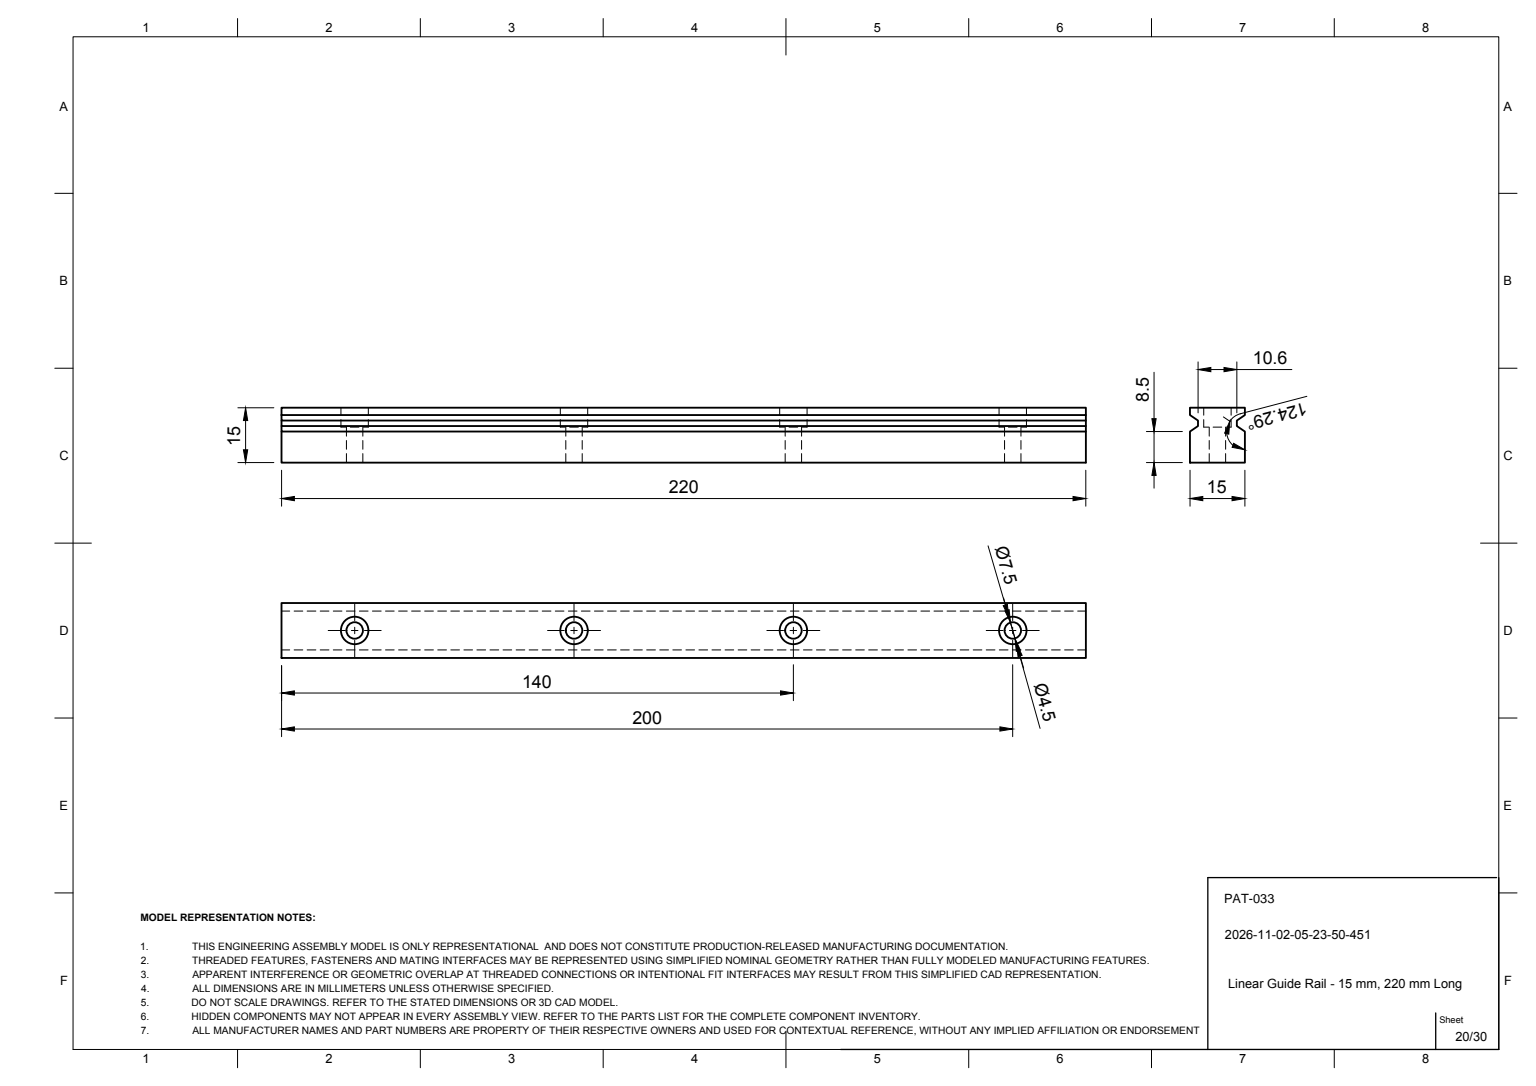
ISO-10303-21;
HEADER;
/* Generated by software containing ST-Developer
 * from STEP Tools, Inc. (www.steptools.com) 
 */

FILE_DESCRIPTION(
/* description */ ('Dual-rail gantry carriage'),
/* implementation_level */ '2;1');

FILE_NAME(
/* name */ 'Linear Guide Rail - 15 mm, 220 mm Long.step',
/* time_stamp */ '2026-10-27T10:49:15-07:00',
/* author */ (''),
/* organization */ (''),
/* preprocessor_version */ 'ST-DEVELOPER v20.2',
/* originating_system */ 'Autodesk Translation Framework v15.17.0.0',
/* authorisation */ '');

FILE_SCHEMA (('AUTOMOTIVE_DESIGN { 1 0 10303 214 3 1 1 }'));
ENDSEC;

DATA;
#10=MECHANICAL_DESIGN_GEOMETRIC_PRESENTATION_REPRESENTATION('',(#600),#12804);
#538=SHAPE_REPRESENTATION_RELATIONSHIP('SRR','None',#13016,#569);
#569=ADVANCED_BREP_SHAPE_REPRESENTATION('',(#631),#12786);
#600=STYLED_ITEM('',(#13240),#631);
#631=MANIFOLD_SOLID_BREP('Body1',#7378);
#692=FACE_BOUND('',#1660,.T.);
#693=FACE_BOUND('',#1663,.T.);
#694=FACE_BOUND('',#1666,.T.);
#695=FACE_BOUND('',#1669,.T.);
#696=FACE_BOUND('',#1679,.T.);
#697=FACE_BOUND('',#1680,.T.);
#698=FACE_BOUND('',#1681,.T.);
#699=FACE_BOUND('',#1682,.T.);
#700=FACE_BOUND('',#1689,.T.);
#701=FACE_BOUND('',#1690,.T.);
#702=FACE_BOUND('',#1691,.T.);
#703=FACE_BOUND('',#1692,.T.);
#902=PLANE('',#7999);
#903=PLANE('',#8004);
#904=PLANE('',#8009);
#905=PLANE('',#8014);
#906=PLANE('',#8024);
#907=PLANE('',#8025);
#908=PLANE('',#8026);
#909=PLANE('',#8027);
#910=PLANE('',#8028);
#911=PLANE('',#8029);
#912=PLANE('',#8030);
#913=PLANE('',#8031);
#914=PLANE('',#8032);
#915=PLANE('',#8033);
#916=PLANE('',#8034);
#917=PLANE('',#8035);
#918=PLANE('',#8036);
#919=PLANE('',#8037);
#1219=FACE_OUTER_BOUND('',#1658,.T.);
#1220=FACE_OUTER_BOUND('',#1659,.T.);
#1221=FACE_OUTER_BOUND('',#1661,.T.);
#1222=FACE_OUTER_BOUND('',#1662,.T.);
#1223=FACE_OUTER_BOUND('',#1664,.T.);
#1224=FACE_OUTER_BOUND('',#1665,.T.);
#1225=FACE_OUTER_BOUND('',#1667,.T.);
#1226=FACE_OUTER_BOUND('',#1668,.T.);
#1227=FACE_OUTER_BOUND('',#1670,.T.);
#1228=FACE_OUTER_BOUND('',#1671,.T.);
#1229=FACE_OUTER_BOUND('',#1672,.T.);
#1230=FACE_OUTER_BOUND('',#1673,.T.);
#1231=FACE_OUTER_BOUND('',#1674,.T.);
#1232=FACE_OUTER_BOUND('',#1675,.T.);
#1233=FACE_OUTER_BOUND('',#1676,.T.);
#1234=FACE_OUTER_BOUND('',#1677,.T.);
#1235=FACE_OUTER_BOUND('',#1678,.T.);
#1236=FACE_OUTER_BOUND('',#1683,.T.);
#1237=FACE_OUTER_BOUND('',#1684,.T.);
#1238=FACE_OUTER_BOUND('',#1685,.T.);
#1239=FACE_OUTER_BOUND('',#1686,.T.);
#1240=FACE_OUTER_BOUND('',#1687,.T.);
#1241=FACE_OUTER_BOUND('',#1688,.T.);
#1242=FACE_OUTER_BOUND('',#1693,.T.);
#1243=FACE_OUTER_BOUND('',#1694,.T.);
#1244=FACE_OUTER_BOUND('',#1695,.T.);
#1658=EDGE_LOOP('',(#5897,#5898,#5899,#5900));
#1659=EDGE_LOOP('',(#5901));
#1660=EDGE_LOOP('',(#5902));
#1661=EDGE_LOOP('',(#5903,#5904,#5905,#5906));
#1662=EDGE_LOOP('',(#5907));
#1663=EDGE_LOOP('',(#5908));
#1664=EDGE_LOOP('',(#5909,#5910,#5911,#5912));
#1665=EDGE_LOOP('',(#5913));
#1666=EDGE_LOOP('',(#5914));
#1667=EDGE_LOOP('',(#5915,#5916,#5917,#5918));
#1668=EDGE_LOOP('',(#5919));
#1669=EDGE_LOOP('',(#5920));
#1670=EDGE_LOOP('',(#5921,#5922,#5923,#5924));
#1671=EDGE_LOOP('',(#5925,#5926,#5927,#5928));
#1672=EDGE_LOOP('',(#5929,#5930,#5931,#5932));
#1673=EDGE_LOOP('',(#5933,#5934,#5935,#5936));
#1674=EDGE_LOOP('',(#5937,#5938,#5939,#5940));
#1675=EDGE_LOOP('',(#5941,#5942,#5943,#5944));
#1676=EDGE_LOOP('',(#5945,#5946,#5947,#5948));
#1677=EDGE_LOOP('',(#5949,#5950,#5951,#5952));
#1678=EDGE_LOOP('',(#5953,#5954,#5955,#5956));
#1679=EDGE_LOOP('',(#5957));
#1680=EDGE_LOOP('',(#5958));
#1681=EDGE_LOOP('',(#5959));
#1682=EDGE_LOOP('',(#5960));
#1683=EDGE_LOOP('',(#5961,#5962,#5963,#5964));
#1684=EDGE_LOOP('',(#5965,#5966,#5967,#5968));
#1685=EDGE_LOOP('',(#5969,#5970,#5971,#5972));
#1686=EDGE_LOOP('',(#5973,#5974,#5975,#5976));
#1687=EDGE_LOOP('',(#5977,#5978,#5979,#5980));
#1688=EDGE_LOOP('',(#5981,#5982,#5983,#5984));
#1689=EDGE_LOOP('',(#5985));
#1690=EDGE_LOOP('',(#5986));
#1691=EDGE_LOOP('',(#5987));
#1692=EDGE_LOOP('',(#5988));
#1693=EDGE_LOOP('',(#5989,#5990,#5991,#5992));
#1694=EDGE_LOOP('',(#5993,#5994,#5995,#5996,#5997,#5998,#5999,#6000,#6001,
#6002,#6003,#6004));
#1695=EDGE_LOOP('',(#6005,#6006,#6007,#6008,#6009,#6010,#6011,#6012,#6013,
#6014,#6015,#6016));
#2297=LINE('',#11562,#3006);
#2298=LINE('',#11571,#3007);
#2299=LINE('',#11580,#3008);
#2300=LINE('',#11589,#3009);
#2301=LINE('',#11597,#3010);
#2302=LINE('',#11601,#3011);
#2303=LINE('',#11605,#3012);
#2304=LINE('',#11609,#3013);
#2305=LINE('',#11613,#3014);
#2306=LINE('',#11615,#3015);
#2307=LINE('',#11617,#3016);
#2308=LINE('',#11618,#3017);
#2309=LINE('',#11621,#3018);
#2310=LINE('',#11623,#3019);
#2311=LINE('',#11624,#3020);
#2312=LINE('',#11627,#3021);
#2313=LINE('',#11629,#3022);
#2314=LINE('',#11630,#3023);
#2315=LINE('',#11633,#3024);
#2316=LINE('',#11635,#3025);
#2317=LINE('',#11636,#3026);
#2318=LINE('',#11639,#3027);
#2319=LINE('',#11641,#3028);
#2320=LINE('',#11642,#3029);
#2321=LINE('',#11645,#3030);
#2322=LINE('',#11647,#3031);
#2323=LINE('',#11648,#3032);
#2324=LINE('',#11651,#3033);
#2325=LINE('',#11653,#3034);
#2326=LINE('',#11654,#3035);
#2327=LINE('',#11657,#3036);
#2328=LINE('',#11659,#3037);
#2329=LINE('',#11660,#3038);
#2330=LINE('',#11663,#3039);
#2331=LINE('',#11665,#3040);
#2332=LINE('',#11666,#3041);
#2333=LINE('',#11669,#3042);
#2334=LINE('',#11671,#3043);
#2335=LINE('',#11672,#3044);
#2336=LINE('',#11675,#3045);
#2337=LINE('',#11677,#3046);
#2338=LINE('',#11678,#3047);
#2339=LINE('',#11680,#3048);
#2340=LINE('',#11681,#3049);
#3006=VECTOR('',#9350,0.375);
#3007=VECTOR('',#9361,0.375);
#3008=VECTOR('',#9372,0.375);
#3009=VECTOR('',#9383,0.375);
#3010=VECTOR('',#9394,0.225);
#3011=VECTOR('',#9399,0.225);
#3012=VECTOR('',#9404,0.225);
#3013=VECTOR('',#9409,0.225000000000001);
#3014=VECTOR('',#9412,1.);
#3015=VECTOR('',#9413,1.);
#3016=VECTOR('',#9414,1.);
#3017=VECTOR('',#9415,1.);
#3018=VECTOR('',#9418,1.);
#3019=VECTOR('',#9419,1.);
#3020=VECTOR('',#9420,1.);
#3021=VECTOR('',#9423,1.);
#3022=VECTOR('',#9424,1.);
#3023=VECTOR('',#9425,1.);
#3024=VECTOR('',#9428,1.);
#3025=VECTOR('',#9429,1.);
#3026=VECTOR('',#9430,1.);
#3027=VECTOR('',#9433,1.);
#3028=VECTOR('',#9434,1.);
#3029=VECTOR('',#9435,1.);
#3030=VECTOR('',#9438,1.);
#3031=VECTOR('',#9439,1.);
#3032=VECTOR('',#9440,1.);
#3033=VECTOR('',#9443,1.);
#3034=VECTOR('',#9444,1.);
#3035=VECTOR('',#9445,1.);
#3036=VECTOR('',#9448,1.);
#3037=VECTOR('',#9449,1.);
#3038=VECTOR('',#9450,1.);
#3039=VECTOR('',#9453,1.);
#3040=VECTOR('',#9454,1.);
#3041=VECTOR('',#9455,1.);
#3042=VECTOR('',#9458,1.);
#3043=VECTOR('',#9459,1.);
#3044=VECTOR('',#9460,1.);
#3045=VECTOR('',#9463,1.);
#3046=VECTOR('',#9464,1.);
#3047=VECTOR('',#9465,1.);
#3048=VECTOR('',#9468,1.);
#3049=VECTOR('',#9469,1.);
#3432=CIRCLE('',#7997,0.375);
#3433=CIRCLE('',#7998,0.375);
#3434=CIRCLE('',#8000,0.225);
#3435=CIRCLE('',#8002,0.375);
#3436=CIRCLE('',#8003,0.375);
#3437=CIRCLE('',#8005,0.225);
#3438=CIRCLE('',#8007,0.375);
#3439=CIRCLE('',#8008,0.375);
#3440=CIRCLE('',#8010,0.225);
#3441=CIRCLE('',#8012,0.375);
#3442=CIRCLE('',#8013,0.375);
#3443=CIRCLE('',#8015,0.225000000000001);
#3444=CIRCLE('',#8017,0.225);
#3445=CIRCLE('',#8019,0.225);
#3446=CIRCLE('',#8021,0.225);
#3447=CIRCLE('',#8023,0.225000000000001);
#3832=VERTEX_POINT('',#11559);
#3833=VERTEX_POINT('',#11561);
#3834=VERTEX_POINT('',#11565);
#3835=VERTEX_POINT('',#11568);
#3836=VERTEX_POINT('',#11570);
#3837=VERTEX_POINT('',#11574);
#3838=VERTEX_POINT('',#11577);
#3839=VERTEX_POINT('',#11579);
#3840=VERTEX_POINT('',#11583);
#3841=VERTEX_POINT('',#11586);
#3842=VERTEX_POINT('',#11588);
#3843=VERTEX_POINT('',#11592);
#3844=VERTEX_POINT('',#11595);
#3845=VERTEX_POINT('',#11599);
#3846=VERTEX_POINT('',#11603);
#3847=VERTEX_POINT('',#11607);
#3848=VERTEX_POINT('',#11611);
#3849=VERTEX_POINT('',#11612);
#3850=VERTEX_POINT('',#11614);
#3851=VERTEX_POINT('',#11616);
#3852=VERTEX_POINT('',#11620);
#3853=VERTEX_POINT('',#11622);
#3854=VERTEX_POINT('',#11626);
#3855=VERTEX_POINT('',#11628);
#3856=VERTEX_POINT('',#11632);
#3857=VERTEX_POINT('',#11634);
#3858=VERTEX_POINT('',#11638);
#3859=VERTEX_POINT('',#11640);
#3860=VERTEX_POINT('',#11644);
#3861=VERTEX_POINT('',#11646);
#3862=VERTEX_POINT('',#11650);
#3863=VERTEX_POINT('',#11652);
#3864=VERTEX_POINT('',#11656);
#3865=VERTEX_POINT('',#11658);
#3866=VERTEX_POINT('',#11662);
#3867=VERTEX_POINT('',#11664);
#3868=VERTEX_POINT('',#11668);
#3869=VERTEX_POINT('',#11670);
#3870=VERTEX_POINT('',#11674);
#3871=VERTEX_POINT('',#11676);
#4571=EDGE_CURVE('',#3832,#3832,#3432,.T.);
#4572=EDGE_CURVE('',#3832,#3833,#2297,.T.);
#4573=EDGE_CURVE('',#3833,#3833,#3433,.T.);
#4574=EDGE_CURVE('',#3834,#3834,#3434,.T.);
#4575=EDGE_CURVE('',#3835,#3835,#3435,.T.);
#4576=EDGE_CURVE('',#3835,#3836,#2298,.T.);
#4577=EDGE_CURVE('',#3836,#3836,#3436,.T.);
#4578=EDGE_CURVE('',#3837,#3837,#3437,.T.);
#4579=EDGE_CURVE('',#3838,#3838,#3438,.T.);
#4580=EDGE_CURVE('',#3838,#3839,#2299,.T.);
#4581=EDGE_CURVE('',#3839,#3839,#3439,.T.);
#4582=EDGE_CURVE('',#3840,#3840,#3440,.T.);
#4583=EDGE_CURVE('',#3841,#3841,#3441,.T.);
#4584=EDGE_CURVE('',#3841,#3842,#2300,.T.);
#4585=EDGE_CURVE('',#3842,#3842,#3442,.T.);
#4586=EDGE_CURVE('',#3843,#3843,#3443,.T.);
#4587=EDGE_CURVE('',#3844,#3844,#3444,.T.);
#4588=EDGE_CURVE('',#3844,#3834,#2301,.T.);
#4589=EDGE_CURVE('',#3845,#3845,#3445,.T.);
#4590=EDGE_CURVE('',#3845,#3837,#2302,.T.);
#4591=EDGE_CURVE('',#3846,#3846,#3446,.T.);
#4592=EDGE_CURVE('',#3846,#3840,#2303,.T.);
#4593=EDGE_CURVE('',#3847,#3847,#3447,.T.);
#4594=EDGE_CURVE('',#3847,#3843,#2304,.T.);
#4595=EDGE_CURVE('',#3848,#3849,#2305,.T.);
#4596=EDGE_CURVE('',#3849,#3850,#2306,.T.);
#4597=EDGE_CURVE('',#3851,#3850,#2307,.T.);
#4598=EDGE_CURVE('',#3848,#3851,#2308,.T.);
#4599=EDGE_CURVE('',#3852,#3848,#2309,.T.);
#4600=EDGE_CURVE('',#3853,#3851,#2310,.T.);
#4601=EDGE_CURVE('',#3852,#3853,#2311,.T.);
#4602=EDGE_CURVE('',#3854,#3852,#2312,.T.);
#4603=EDGE_CURVE('',#3855,#3853,#2313,.T.);
#4604=EDGE_CURVE('',#3854,#3855,#2314,.T.);
#4605=EDGE_CURVE('',#3856,#3854,#2315,.T.);
#4606=EDGE_CURVE('',#3857,#3855,#2316,.T.);
#4607=EDGE_CURVE('',#3856,#3857,#2317,.T.);
#4608=EDGE_CURVE('',#3858,#3856,#2318,.T.);
#4609=EDGE_CURVE('',#3859,#3857,#2319,.T.);
#4610=EDGE_CURVE('',#3858,#3859,#2320,.T.);
#4611=EDGE_CURVE('',#3860,#3858,#2321,.T.);
#4612=EDGE_CURVE('',#3861,#3859,#2322,.T.);
#4613=EDGE_CURVE('',#3860,#3861,#2323,.T.);
#4614=EDGE_CURVE('',#3862,#3860,#2324,.T.);
#4615=EDGE_CURVE('',#3863,#3861,#2325,.T.);
#4616=EDGE_CURVE('',#3862,#3863,#2326,.T.);
#4617=EDGE_CURVE('',#3864,#3862,#2327,.T.);
#4618=EDGE_CURVE('',#3865,#3863,#2328,.T.);
#4619=EDGE_CURVE('',#3864,#3865,#2329,.T.);
#4620=EDGE_CURVE('',#3866,#3864,#2330,.T.);
#4621=EDGE_CURVE('',#3867,#3865,#2331,.T.);
#4622=EDGE_CURVE('',#3866,#3867,#2332,.T.);
#4623=EDGE_CURVE('',#3868,#3866,#2333,.T.);
#4624=EDGE_CURVE('',#3869,#3867,#2334,.T.);
#4625=EDGE_CURVE('',#3868,#3869,#2335,.T.);
#4626=EDGE_CURVE('',#3870,#3868,#2336,.T.);
#4627=EDGE_CURVE('',#3871,#3869,#2337,.T.);
#4628=EDGE_CURVE('',#3870,#3871,#2338,.T.);
#4629=EDGE_CURVE('',#3849,#3870,#2339,.T.);
#4630=EDGE_CURVE('',#3850,#3871,#2340,.T.);
#5897=ORIENTED_EDGE('',*,*,#4571,.F.);
#5898=ORIENTED_EDGE('',*,*,#4572,.T.);
#5899=ORIENTED_EDGE('',*,*,#4573,.F.);
#5900=ORIENTED_EDGE('',*,*,#4572,.F.);
#5901=ORIENTED_EDGE('',*,*,#4571,.T.);
#5902=ORIENTED_EDGE('',*,*,#4574,.F.);
#5903=ORIENTED_EDGE('',*,*,#4575,.F.);
#5904=ORIENTED_EDGE('',*,*,#4576,.T.);
#5905=ORIENTED_EDGE('',*,*,#4577,.F.);
#5906=ORIENTED_EDGE('',*,*,#4576,.F.);
#5907=ORIENTED_EDGE('',*,*,#4575,.T.);
#5908=ORIENTED_EDGE('',*,*,#4578,.F.);
#5909=ORIENTED_EDGE('',*,*,#4579,.F.);
#5910=ORIENTED_EDGE('',*,*,#4580,.T.);
#5911=ORIENTED_EDGE('',*,*,#4581,.F.);
#5912=ORIENTED_EDGE('',*,*,#4580,.F.);
#5913=ORIENTED_EDGE('',*,*,#4579,.T.);
#5914=ORIENTED_EDGE('',*,*,#4582,.F.);
#5915=ORIENTED_EDGE('',*,*,#4583,.F.);
#5916=ORIENTED_EDGE('',*,*,#4584,.T.);
#5917=ORIENTED_EDGE('',*,*,#4585,.F.);
#5918=ORIENTED_EDGE('',*,*,#4584,.F.);
#5919=ORIENTED_EDGE('',*,*,#4583,.T.);
#5920=ORIENTED_EDGE('',*,*,#4586,.F.);
#5921=ORIENTED_EDGE('',*,*,#4587,.F.);
#5922=ORIENTED_EDGE('',*,*,#4588,.T.);
#5923=ORIENTED_EDGE('',*,*,#4574,.T.);
#5924=ORIENTED_EDGE('',*,*,#4588,.F.);
#5925=ORIENTED_EDGE('',*,*,#4589,.F.);
#5926=ORIENTED_EDGE('',*,*,#4590,.T.);
#5927=ORIENTED_EDGE('',*,*,#4578,.T.);
#5928=ORIENTED_EDGE('',*,*,#4590,.F.);
#5929=ORIENTED_EDGE('',*,*,#4591,.F.);
#5930=ORIENTED_EDGE('',*,*,#4592,.T.);
#5931=ORIENTED_EDGE('',*,*,#4582,.T.);
#5932=ORIENTED_EDGE('',*,*,#4592,.F.);
#5933=ORIENTED_EDGE('',*,*,#4593,.F.);
#5934=ORIENTED_EDGE('',*,*,#4594,.T.);
#5935=ORIENTED_EDGE('',*,*,#4586,.T.);
#5936=ORIENTED_EDGE('',*,*,#4594,.F.);
#5937=ORIENTED_EDGE('',*,*,#4595,.T.);
#5938=ORIENTED_EDGE('',*,*,#4596,.T.);
#5939=ORIENTED_EDGE('',*,*,#4597,.F.);
#5940=ORIENTED_EDGE('',*,*,#4598,.F.);
#5941=ORIENTED_EDGE('',*,*,#4599,.T.);
#5942=ORIENTED_EDGE('',*,*,#4598,.T.);
#5943=ORIENTED_EDGE('',*,*,#4600,.F.);
#5944=ORIENTED_EDGE('',*,*,#4601,.F.);
#5945=ORIENTED_EDGE('',*,*,#4602,.T.);
#5946=ORIENTED_EDGE('',*,*,#4601,.T.);
#5947=ORIENTED_EDGE('',*,*,#4603,.F.);
#5948=ORIENTED_EDGE('',*,*,#4604,.F.);
#5949=ORIENTED_EDGE('',*,*,#4605,.T.);
#5950=ORIENTED_EDGE('',*,*,#4604,.T.);
#5951=ORIENTED_EDGE('',*,*,#4606,.F.);
#5952=ORIENTED_EDGE('',*,*,#4607,.F.);
#5953=ORIENTED_EDGE('',*,*,#4608,.T.);
#5954=ORIENTED_EDGE('',*,*,#4607,.T.);
#5955=ORIENTED_EDGE('',*,*,#4609,.F.);
#5956=ORIENTED_EDGE('',*,*,#4610,.F.);
#5957=ORIENTED_EDGE('',*,*,#4585,.T.);
#5958=ORIENTED_EDGE('',*,*,#4581,.T.);
#5959=ORIENTED_EDGE('',*,*,#4577,.T.);
#5960=ORIENTED_EDGE('',*,*,#4573,.T.);
#5961=ORIENTED_EDGE('',*,*,#4611,.T.);
#5962=ORIENTED_EDGE('',*,*,#4610,.T.);
#5963=ORIENTED_EDGE('',*,*,#4612,.F.);
#5964=ORIENTED_EDGE('',*,*,#4613,.F.);
#5965=ORIENTED_EDGE('',*,*,#4614,.T.);
#5966=ORIENTED_EDGE('',*,*,#4613,.T.);
#5967=ORIENTED_EDGE('',*,*,#4615,.F.);
#5968=ORIENTED_EDGE('',*,*,#4616,.F.);
#5969=ORIENTED_EDGE('',*,*,#4617,.T.);
#5970=ORIENTED_EDGE('',*,*,#4616,.T.);
#5971=ORIENTED_EDGE('',*,*,#4618,.F.);
#5972=ORIENTED_EDGE('',*,*,#4619,.F.);
#5973=ORIENTED_EDGE('',*,*,#4620,.T.);
#5974=ORIENTED_EDGE('',*,*,#4619,.T.);
#5975=ORIENTED_EDGE('',*,*,#4621,.F.);
#5976=ORIENTED_EDGE('',*,*,#4622,.F.);
#5977=ORIENTED_EDGE('',*,*,#4623,.T.);
#5978=ORIENTED_EDGE('',*,*,#4622,.T.);
#5979=ORIENTED_EDGE('',*,*,#4624,.F.);
#5980=ORIENTED_EDGE('',*,*,#4625,.F.);
#5981=ORIENTED_EDGE('',*,*,#4626,.T.);
#5982=ORIENTED_EDGE('',*,*,#4625,.T.);
#5983=ORIENTED_EDGE('',*,*,#4627,.F.);
#5984=ORIENTED_EDGE('',*,*,#4628,.F.);
#5985=ORIENTED_EDGE('',*,*,#4587,.T.);
#5986=ORIENTED_EDGE('',*,*,#4589,.T.);
#5987=ORIENTED_EDGE('',*,*,#4591,.T.);
#5988=ORIENTED_EDGE('',*,*,#4593,.T.);
#5989=ORIENTED_EDGE('',*,*,#4629,.T.);
#5990=ORIENTED_EDGE('',*,*,#4628,.T.);
#5991=ORIENTED_EDGE('',*,*,#4630,.F.);
#5992=ORIENTED_EDGE('',*,*,#4596,.F.);
#5993=ORIENTED_EDGE('',*,*,#4630,.T.);
#5994=ORIENTED_EDGE('',*,*,#4627,.T.);
#5995=ORIENTED_EDGE('',*,*,#4624,.T.);
#5996=ORIENTED_EDGE('',*,*,#4621,.T.);
#5997=ORIENTED_EDGE('',*,*,#4618,.T.);
#5998=ORIENTED_EDGE('',*,*,#4615,.T.);
#5999=ORIENTED_EDGE('',*,*,#4612,.T.);
#6000=ORIENTED_EDGE('',*,*,#4609,.T.);
#6001=ORIENTED_EDGE('',*,*,#4606,.T.);
#6002=ORIENTED_EDGE('',*,*,#4603,.T.);
#6003=ORIENTED_EDGE('',*,*,#4600,.T.);
#6004=ORIENTED_EDGE('',*,*,#4597,.T.);
#6005=ORIENTED_EDGE('',*,*,#4629,.F.);
#6006=ORIENTED_EDGE('',*,*,#4595,.F.);
#6007=ORIENTED_EDGE('',*,*,#4599,.F.);
#6008=ORIENTED_EDGE('',*,*,#4602,.F.);
#6009=ORIENTED_EDGE('',*,*,#4605,.F.);
#6010=ORIENTED_EDGE('',*,*,#4608,.F.);
#6011=ORIENTED_EDGE('',*,*,#4611,.F.);
#6012=ORIENTED_EDGE('',*,*,#4614,.F.);
#6013=ORIENTED_EDGE('',*,*,#4617,.F.);
#6014=ORIENTED_EDGE('',*,*,#4620,.F.);
#6015=ORIENTED_EDGE('',*,*,#4623,.F.);
#6016=ORIENTED_EDGE('',*,*,#4626,.F.);
#6922=CYLINDRICAL_SURFACE('',#7996,0.375);
#6923=CYLINDRICAL_SURFACE('',#8001,0.375);
#6924=CYLINDRICAL_SURFACE('',#8006,0.375);
#6925=CYLINDRICAL_SURFACE('',#8011,0.375);
#6926=CYLINDRICAL_SURFACE('',#8016,0.225);
#6927=CYLINDRICAL_SURFACE('',#8018,0.225);
#6928=CYLINDRICAL_SURFACE('',#8020,0.225);
#6929=CYLINDRICAL_SURFACE('',#8022,0.225000000000001);
#7145=ADVANCED_FACE('',(#1219),#6922,.F.);
#7146=ADVANCED_FACE('',(#1220,#692),#902,.T.);
#7147=ADVANCED_FACE('',(#1221),#6923,.F.);
#7148=ADVANCED_FACE('',(#1222,#693),#903,.T.);
#7149=ADVANCED_FACE('',(#1223),#6924,.F.);
#7150=ADVANCED_FACE('',(#1224,#694),#904,.T.);
#7151=ADVANCED_FACE('',(#1225),#6925,.F.);
#7152=ADVANCED_FACE('',(#1226,#695),#905,.T.);
#7153=ADVANCED_FACE('',(#1227),#6926,.F.);
#7154=ADVANCED_FACE('',(#1228),#6927,.F.);
#7155=ADVANCED_FACE('',(#1229),#6928,.F.);
#7156=ADVANCED_FACE('',(#1230),#6929,.F.);
#7157=ADVANCED_FACE('',(#1231),#906,.T.);
#7158=ADVANCED_FACE('',(#1232),#907,.T.);
#7159=ADVANCED_FACE('',(#1233),#908,.T.);
#7160=ADVANCED_FACE('',(#1234),#909,.T.);
#7161=ADVANCED_FACE('',(#1235,#696,#697,#698,#699),#910,.T.);
#7162=ADVANCED_FACE('',(#1236),#911,.T.);
#7163=ADVANCED_FACE('',(#1237),#912,.T.);
#7164=ADVANCED_FACE('',(#1238),#913,.T.);
#7165=ADVANCED_FACE('',(#1239),#914,.T.);
#7166=ADVANCED_FACE('',(#1240),#915,.T.);
#7167=ADVANCED_FACE('',(#1241,#700,#701,#702,#703),#916,.T.);
#7168=ADVANCED_FACE('',(#1242),#917,.T.);
#7169=ADVANCED_FACE('',(#1243),#918,.T.);
#7170=ADVANCED_FACE('',(#1244),#919,.F.);
#7378=CLOSED_SHELL('',(#7145,#7146,#7147,#7148,#7149,#7150,#7151,#7152,
#7153,#7154,#7155,#7156,#7157,#7158,#7159,#7160,#7161,#7162,#7163,#7164,
#7165,#7166,#7167,#7168,#7169,#7170));
#7995=AXIS2_PLACEMENT_3D('',#11557,#9344,#9345);
#7996=AXIS2_PLACEMENT_3D('',#11558,#9346,#9347);
#7997=AXIS2_PLACEMENT_3D('',#11560,#9348,#9349);
#7998=AXIS2_PLACEMENT_3D('',#11563,#9351,#9352);
#7999=AXIS2_PLACEMENT_3D('',#11564,#9353,#9354);
#8000=AXIS2_PLACEMENT_3D('',#11566,#9355,#9356);
#8001=AXIS2_PLACEMENT_3D('',#11567,#9357,#9358);
#8002=AXIS2_PLACEMENT_3D('',#11569,#9359,#9360);
#8003=AXIS2_PLACEMENT_3D('',#11572,#9362,#9363);
#8004=AXIS2_PLACEMENT_3D('',#11573,#9364,#9365);
#8005=AXIS2_PLACEMENT_3D('',#11575,#9366,#9367);
#8006=AXIS2_PLACEMENT_3D('',#11576,#9368,#9369);
#8007=AXIS2_PLACEMENT_3D('',#11578,#9370,#9371);
#8008=AXIS2_PLACEMENT_3D('',#11581,#9373,#9374);
#8009=AXIS2_PLACEMENT_3D('',#11582,#9375,#9376);
#8010=AXIS2_PLACEMENT_3D('',#11584,#9377,#9378);
#8011=AXIS2_PLACEMENT_3D('',#11585,#9379,#9380);
#8012=AXIS2_PLACEMENT_3D('',#11587,#9381,#9382);
#8013=AXIS2_PLACEMENT_3D('',#11590,#9384,#9385);
#8014=AXIS2_PLACEMENT_3D('',#11591,#9386,#9387);
#8015=AXIS2_PLACEMENT_3D('',#11593,#9388,#9389);
#8016=AXIS2_PLACEMENT_3D('',#11594,#9390,#9391);
#8017=AXIS2_PLACEMENT_3D('',#11596,#9392,#9393);
#8018=AXIS2_PLACEMENT_3D('',#11598,#9395,#9396);
#8019=AXIS2_PLACEMENT_3D('',#11600,#9397,#9398);
#8020=AXIS2_PLACEMENT_3D('',#11602,#9400,#9401);
#8021=AXIS2_PLACEMENT_3D('',#11604,#9402,#9403);
#8022=AXIS2_PLACEMENT_3D('',#11606,#9405,#9406);
#8023=AXIS2_PLACEMENT_3D('',#11608,#9407,#9408);
#8024=AXIS2_PLACEMENT_3D('',#11610,#9410,#9411);
#8025=AXIS2_PLACEMENT_3D('',#11619,#9416,#9417);
#8026=AXIS2_PLACEMENT_3D('',#11625,#9421,#9422);
#8027=AXIS2_PLACEMENT_3D('',#11631,#9426,#9427);
#8028=AXIS2_PLACEMENT_3D('',#11637,#9431,#9432);
#8029=AXIS2_PLACEMENT_3D('',#11643,#9436,#9437);
#8030=AXIS2_PLACEMENT_3D('',#11649,#9441,#9442);
#8031=AXIS2_PLACEMENT_3D('',#11655,#9446,#9447);
#8032=AXIS2_PLACEMENT_3D('',#11661,#9451,#9452);
#8033=AXIS2_PLACEMENT_3D('',#11667,#9456,#9457);
#8034=AXIS2_PLACEMENT_3D('',#11673,#9461,#9462);
#8035=AXIS2_PLACEMENT_3D('',#11679,#9466,#9467);
#8036=AXIS2_PLACEMENT_3D('',#11682,#9470,#9471);
#8037=AXIS2_PLACEMENT_3D('',#11683,#9472,#9473);
#9344=DIRECTION('axis',(0.,0.,1.));
#9345=DIRECTION('refdir',(1.,0.,0.));
#9346=DIRECTION('center_axis',(0.,0.,1.));
#9347=DIRECTION('ref_axis',(1.,0.,0.));
#9348=DIRECTION('center_axis',(0.,0.,1.));
#9349=DIRECTION('ref_axis',(1.,0.,0.));
#9350=DIRECTION('',(0.,0.,1.));
#9351=DIRECTION('center_axis',(0.,0.,-1.));
#9352=DIRECTION('ref_axis',(1.,0.,0.));
#9353=DIRECTION('center_axis',(0.,0.,1.));
#9354=DIRECTION('ref_axis',(1.,0.,0.));
#9355=DIRECTION('center_axis',(0.,0.,1.));
#9356=DIRECTION('ref_axis',(1.,0.,0.));
#9357=DIRECTION('center_axis',(0.,0.,1.));
#9358=DIRECTION('ref_axis',(1.,0.,0.));
#9359=DIRECTION('center_axis',(0.,0.,1.));
#9360=DIRECTION('ref_axis',(1.,0.,0.));
#9361=DIRECTION('',(0.,0.,1.));
#9362=DIRECTION('center_axis',(0.,0.,-1.));
#9363=DIRECTION('ref_axis',(1.,0.,0.));
#9364=DIRECTION('center_axis',(0.,0.,1.));
#9365=DIRECTION('ref_axis',(1.,0.,0.));
#9366=DIRECTION('center_axis',(0.,0.,1.));
#9367=DIRECTION('ref_axis',(1.,0.,0.));
#9368=DIRECTION('center_axis',(0.,0.,1.));
#9369=DIRECTION('ref_axis',(1.,0.,0.));
#9370=DIRECTION('center_axis',(0.,0.,1.));
#9371=DIRECTION('ref_axis',(1.,0.,0.));
#9372=DIRECTION('',(0.,0.,1.));
#9373=DIRECTION('center_axis',(0.,0.,-1.));
#9374=DIRECTION('ref_axis',(1.,0.,0.));
#9375=DIRECTION('center_axis',(0.,0.,1.));
#9376=DIRECTION('ref_axis',(1.,0.,0.));
#9377=DIRECTION('center_axis',(0.,0.,1.));
#9378=DIRECTION('ref_axis',(1.,0.,0.));
#9379=DIRECTION('center_axis',(0.,0.,1.));
#9380=DIRECTION('ref_axis',(1.,0.,0.));
#9381=DIRECTION('center_axis',(0.,0.,1.));
#9382=DIRECTION('ref_axis',(1.,0.,0.));
#9383=DIRECTION('',(0.,0.,1.));
#9384=DIRECTION('center_axis',(0.,0.,-1.));
#9385=DIRECTION('ref_axis',(1.,0.,0.));
#9386=DIRECTION('center_axis',(0.,0.,1.));
#9387=DIRECTION('ref_axis',(1.,0.,0.));
#9388=DIRECTION('center_axis',(0.,0.,1.));
#9389=DIRECTION('ref_axis',(1.,0.,0.));
#9390=DIRECTION('center_axis',(0.,0.,1.));
#9391=DIRECTION('ref_axis',(1.,0.,0.));
#9392=DIRECTION('center_axis',(0.,0.,1.));
#9393=DIRECTION('ref_axis',(1.,0.,0.));
#9394=DIRECTION('',(0.,0.,1.));
#9395=DIRECTION('center_axis',(0.,0.,1.));
#9396=DIRECTION('ref_axis',(1.,0.,0.));
#9397=DIRECTION('center_axis',(0.,0.,1.));
#9398=DIRECTION('ref_axis',(1.,0.,0.));
#9399=DIRECTION('',(0.,0.,1.));
#9400=DIRECTION('center_axis',(0.,0.,1.));
#9401=DIRECTION('ref_axis',(1.,0.,0.));
#9402=DIRECTION('center_axis',(0.,0.,1.));
#9403=DIRECTION('ref_axis',(1.,0.,0.));
#9404=DIRECTION('',(0.,0.,1.));
#9405=DIRECTION('center_axis',(0.,0.,1.));
#9406=DIRECTION('ref_axis',(1.,0.,0.));
#9407=DIRECTION('center_axis',(0.,0.,1.));
#9408=DIRECTION('ref_axis',(1.,0.,0.));
#9409=DIRECTION('',(0.,0.,1.));
#9410=DIRECTION('center_axis',(0.,-0.56333682464151,0.826227342807548));
#9411=DIRECTION('ref_axis',(0.,-0.826227342807548,-0.56333682464151));
#9412=DIRECTION('',(0.,-0.826227342807548,-0.56333682464151));
#9413=DIRECTION('',(1.,0.,0.));
#9414=DIRECTION('',(0.,-0.826227342807548,-0.56333682464151));
#9415=DIRECTION('',(1.,0.,0.));
#9416=DIRECTION('center_axis',(0.,-1.,0.));
#9417=DIRECTION('ref_axis',(0.,0.,-1.));
#9418=DIRECTION('',(0.,0.,-1.));
#9419=DIRECTION('',(0.,0.,-1.));
#9420=DIRECTION('',(1.,0.,0.));
#9421=DIRECTION('center_axis',(0.,-0.56333682464151,-0.826227342807548));
#9422=DIRECTION('ref_axis',(0.,0.826227342807548,-0.56333682464151));
#9423=DIRECTION('',(0.,0.826227342807548,-0.56333682464151));
#9424=DIRECTION('',(0.,0.826227342807548,-0.56333682464151));
#9425=DIRECTION('',(1.,0.,0.));
#9426=DIRECTION('center_axis',(0.,-1.,0.));
#9427=DIRECTION('ref_axis',(0.,0.,-1.));
#9428=DIRECTION('',(0.,0.,-1.));
#9429=DIRECTION('',(0.,0.,-1.));
#9430=DIRECTION('',(1.,0.,0.));
#9431=DIRECTION('center_axis',(0.,0.,1.));
#9432=DIRECTION('ref_axis',(0.,-1.,0.));
#9433=DIRECTION('',(0.,-1.,0.));
#9434=DIRECTION('',(0.,-1.,0.));
#9435=DIRECTION('',(1.,0.,0.));
#9436=DIRECTION('center_axis',(0.,1.,0.));
#9437=DIRECTION('ref_axis',(0.,0.,1.));
#9438=DIRECTION('',(0.,0.,1.));
#9439=DIRECTION('',(0.,0.,1.));
#9440=DIRECTION('',(1.,0.,0.));
#9441=DIRECTION('center_axis',(0.,0.56333682464151,-0.826227342807548));
#9442=DIRECTION('ref_axis',(0.,0.826227342807548,0.56333682464151));
#9443=DIRECTION('',(0.,0.826227342807548,0.56333682464151));
#9444=DIRECTION('',(0.,0.826227342807548,0.56333682464151));
#9445=DIRECTION('',(1.,0.,0.));
#9446=DIRECTION('center_axis',(0.,1.,0.));
#9447=DIRECTION('ref_axis',(0.,0.,1.));
#9448=DIRECTION('',(0.,0.,1.));
#9449=DIRECTION('',(0.,0.,1.));
#9450=DIRECTION('',(1.,0.,0.));
#9451=DIRECTION('center_axis',(0.,0.56333682464151,0.826227342807548));
#9452=DIRECTION('ref_axis',(0.,-0.826227342807548,0.56333682464151));
#9453=DIRECTION('',(0.,-0.826227342807548,0.56333682464151));
#9454=DIRECTION('',(0.,-0.826227342807548,0.56333682464151));
#9455=DIRECTION('',(1.,0.,0.));
#9456=DIRECTION('center_axis',(0.,1.,0.));
#9457=DIRECTION('ref_axis',(0.,0.,1.));
#9458=DIRECTION('',(0.,0.,1.));
#9459=DIRECTION('',(0.,0.,1.));
#9460=DIRECTION('',(1.,0.,0.));
#9461=DIRECTION('center_axis',(0.,0.,-1.));
#9462=DIRECTION('ref_axis',(0.,1.,0.));
#9463=DIRECTION('',(0.,1.,0.));
#9464=DIRECTION('',(0.,1.,0.));
#9465=DIRECTION('',(1.,0.,0.));
#9466=DIRECTION('center_axis',(0.,-1.,0.));
#9467=DIRECTION('ref_axis',(0.,0.,-1.));
#9468=DIRECTION('',(0.,0.,-1.));
#9469=DIRECTION('',(0.,0.,-1.));
#9470=DIRECTION('center_axis',(1.,0.,0.));
#9471=DIRECTION('ref_axis',(0.,0.,-1.));
#9472=DIRECTION('center_axis',(1.,0.,0.));
#9473=DIRECTION('ref_axis',(0.,0.,-1.));
#11557=CARTESIAN_POINT('',(0.,0.,0.));
#11558=CARTESIAN_POINT('Origin',(14.,0.,0.97));
#11559=CARTESIAN_POINT('',(13.625,-4.59242549680257E-17,0.97));
#11560=CARTESIAN_POINT('Origin',(14.,0.,0.97));
#11561=CARTESIAN_POINT('',(13.625,4.59242549680257E-17,1.5));
#11562=CARTESIAN_POINT('',(13.625,-4.59242549680257E-17,0.97));
#11563=CARTESIAN_POINT('Origin',(14.,0.,1.5));
#11564=CARTESIAN_POINT('Origin',(14.,0.,0.97));
#11565=CARTESIAN_POINT('',(13.775,-2.75545529808154E-17,0.97));
#11566=CARTESIAN_POINT('Origin',(14.,0.,0.97));
#11567=CARTESIAN_POINT('Origin',(8.,0.,0.97));
#11568=CARTESIAN_POINT('',(7.625,-4.59242549680257E-17,0.97));
#11569=CARTESIAN_POINT('Origin',(8.,0.,0.97));
#11570=CARTESIAN_POINT('',(7.625,4.59242549680257E-17,1.5));
#11571=CARTESIAN_POINT('',(7.625,-4.59242549680257E-17,0.97));
#11572=CARTESIAN_POINT('Origin',(8.,0.,1.5));
#11573=CARTESIAN_POINT('Origin',(8.,0.,0.97));
#11574=CARTESIAN_POINT('',(7.775,-2.75545529808154E-17,0.97));
#11575=CARTESIAN_POINT('Origin',(8.,0.,0.97));
#11576=CARTESIAN_POINT('Origin',(2.,0.,0.97));
#11577=CARTESIAN_POINT('',(1.625,-4.59242549680257E-17,0.97));
#11578=CARTESIAN_POINT('Origin',(2.,0.,0.97));
#11579=CARTESIAN_POINT('',(1.625,4.59242549680257E-17,1.5));
#11580=CARTESIAN_POINT('',(1.625,-4.59242549680257E-17,0.97));
#11581=CARTESIAN_POINT('Origin',(2.,0.,1.5));
#11582=CARTESIAN_POINT('Origin',(2.,0.,0.97));
#11583=CARTESIAN_POINT('',(1.775,-2.75545529808155E-17,0.97));
#11584=CARTESIAN_POINT('Origin',(2.,0.,0.97));
#11585=CARTESIAN_POINT('Origin',(20.,0.,0.97));
#11586=CARTESIAN_POINT('',(19.625,-4.59242549680257E-17,0.97));
#11587=CARTESIAN_POINT('Origin',(20.,0.,0.97));
#11588=CARTESIAN_POINT('',(19.625,4.59242549680257E-17,1.5));
#11589=CARTESIAN_POINT('',(19.625,-4.59242549680257E-17,0.97));
#11590=CARTESIAN_POINT('Origin',(20.,0.,1.5));
#11591=CARTESIAN_POINT('Origin',(20.,0.,0.97));
#11592=CARTESIAN_POINT('',(19.775,-2.75545529808156E-17,0.97));
#11593=CARTESIAN_POINT('Origin',(20.,0.,0.97));
#11594=CARTESIAN_POINT('Origin',(14.,0.,-0.1));
#11595=CARTESIAN_POINT('',(13.775,-2.75545529808154E-17,0.));
#11596=CARTESIAN_POINT('Origin',(14.,0.,0.));
#11597=CARTESIAN_POINT('',(13.775,-2.75545529808154E-17,-0.1));
#11598=CARTESIAN_POINT('Origin',(8.,0.,-0.1));
#11599=CARTESIAN_POINT('',(7.775,-2.75545529808154E-17,0.));
#11600=CARTESIAN_POINT('Origin',(8.,0.,0.));
#11601=CARTESIAN_POINT('',(7.775,-2.75545529808154E-17,-0.1));
#11602=CARTESIAN_POINT('Origin',(2.,0.,-0.1));
#11603=CARTESIAN_POINT('',(1.775,-2.75545529808155E-17,0.));
#11604=CARTESIAN_POINT('Origin',(2.,0.,0.));
#11605=CARTESIAN_POINT('',(1.775,-2.75545529808155E-17,-0.1));
#11606=CARTESIAN_POINT('Origin',(20.,0.,-0.1));
#11607=CARTESIAN_POINT('',(19.775,-2.75545529808156E-17,0.));
#11608=CARTESIAN_POINT('Origin',(20.,0.,0.));
#11609=CARTESIAN_POINT('',(19.775,-2.75545529808156E-17,-0.1));
#11610=CARTESIAN_POINT('Origin',(0.,-0.53,1.));
#11611=CARTESIAN_POINT('',(0.,-0.53,1.));
#11612=CARTESIAN_POINT('',(0.,-0.75,0.85));
#11613=CARTESIAN_POINT('',(0.,-0.53,1.));
#11614=CARTESIAN_POINT('',(22.,-0.75,0.85));
#11615=CARTESIAN_POINT('',(0.,-0.75,0.85));
#11616=CARTESIAN_POINT('',(22.,-0.53,1.));
#11617=CARTESIAN_POINT('',(22.,-0.53,1.));
#11618=CARTESIAN_POINT('',(0.,-0.53,1.));
#11619=CARTESIAN_POINT('Origin',(0.,-0.53,1.15));
#11620=CARTESIAN_POINT('',(0.,-0.53,1.15));
#11621=CARTESIAN_POINT('',(0.,-0.53,1.15));
#11622=CARTESIAN_POINT('',(22.,-0.53,1.15));
#11623=CARTESIAN_POINT('',(22.,-0.53,1.15));
#11624=CARTESIAN_POINT('',(0.,-0.53,1.15));
#11625=CARTESIAN_POINT('Origin',(0.,-0.75,1.3));
#11626=CARTESIAN_POINT('',(0.,-0.75,1.3));
#11627=CARTESIAN_POINT('',(0.,-0.75,1.3));
#11628=CARTESIAN_POINT('',(22.,-0.75,1.3));
#11629=CARTESIAN_POINT('',(22.,-0.75,1.3));
#11630=CARTESIAN_POINT('',(0.,-0.75,1.3));
#11631=CARTESIAN_POINT('Origin',(0.,-0.75,1.5));
#11632=CARTESIAN_POINT('',(0.,-0.75,1.5));
#11633=CARTESIAN_POINT('',(0.,-0.75,1.5));
#11634=CARTESIAN_POINT('',(22.,-0.75,1.5));
#11635=CARTESIAN_POINT('',(22.,-0.75,1.5));
#11636=CARTESIAN_POINT('',(0.,-0.75,1.5));
#11637=CARTESIAN_POINT('Origin',(0.,0.75,1.5));
#11638=CARTESIAN_POINT('',(0.,0.75,1.5));
#11639=CARTESIAN_POINT('',(0.,0.75,1.5));
#11640=CARTESIAN_POINT('',(22.,0.75,1.5));
#11641=CARTESIAN_POINT('',(22.,0.75,1.5));
#11642=CARTESIAN_POINT('',(0.,0.75,1.5));
#11643=CARTESIAN_POINT('Origin',(0.,0.75,1.3));
#11644=CARTESIAN_POINT('',(0.,0.75,1.3));
#11645=CARTESIAN_POINT('',(0.,0.75,1.3));
#11646=CARTESIAN_POINT('',(22.,0.75,1.3));
#11647=CARTESIAN_POINT('',(22.,0.75,1.3));
#11648=CARTESIAN_POINT('',(0.,0.75,1.3));
#11649=CARTESIAN_POINT('Origin',(0.,0.53,1.15));
#11650=CARTESIAN_POINT('',(0.,0.53,1.15));
#11651=CARTESIAN_POINT('',(0.,0.53,1.15));
#11652=CARTESIAN_POINT('',(22.,0.53,1.15));
#11653=CARTESIAN_POINT('',(22.,0.53,1.15));
#11654=CARTESIAN_POINT('',(0.,0.53,1.15));
#11655=CARTESIAN_POINT('Origin',(0.,0.53,1.));
#11656=CARTESIAN_POINT('',(0.,0.53,1.));
#11657=CARTESIAN_POINT('',(0.,0.53,1.));
#11658=CARTESIAN_POINT('',(22.,0.53,1.));
#11659=CARTESIAN_POINT('',(22.,0.53,1.));
#11660=CARTESIAN_POINT('',(0.,0.53,1.));
#11661=CARTESIAN_POINT('Origin',(0.,0.75,0.85));
#11662=CARTESIAN_POINT('',(0.,0.75,0.85));
#11663=CARTESIAN_POINT('',(0.,0.75,0.85));
#11664=CARTESIAN_POINT('',(22.,0.75,0.85));
#11665=CARTESIAN_POINT('',(22.,0.75,0.85));
#11666=CARTESIAN_POINT('',(0.,0.75,0.85));
#11667=CARTESIAN_POINT('Origin',(0.,0.75,0.));
#11668=CARTESIAN_POINT('',(0.,0.75,0.));
#11669=CARTESIAN_POINT('',(0.,0.75,0.));
#11670=CARTESIAN_POINT('',(22.,0.75,0.));
#11671=CARTESIAN_POINT('',(22.,0.75,0.));
#11672=CARTESIAN_POINT('',(0.,0.75,0.));
#11673=CARTESIAN_POINT('Origin',(0.,-0.75,0.));
#11674=CARTESIAN_POINT('',(0.,-0.75,0.));
#11675=CARTESIAN_POINT('',(0.,-0.75,0.));
#11676=CARTESIAN_POINT('',(22.,-0.75,0.));
#11677=CARTESIAN_POINT('',(22.,-0.75,0.));
#11678=CARTESIAN_POINT('',(0.,-0.75,0.));
#11679=CARTESIAN_POINT('Origin',(0.,-0.75,0.85));
#11680=CARTESIAN_POINT('',(0.,-0.75,0.85));
#11681=CARTESIAN_POINT('',(22.,-0.75,0.85));
#11682=CARTESIAN_POINT('Origin',(22.,0.,0.75));
#11683=CARTESIAN_POINT('Origin',(0.,0.,0.75));
#12750=UNCERTAINTY_MEASURE_WITH_UNIT(LENGTH_MEASURE(0.001),#12805,
'DISTANCE_ACCURACY_VALUE',
'Maximum model space distance between geometric entities at asserted c
onnectivities');
#12768=UNCERTAINTY_MEASURE_WITH_UNIT(LENGTH_MEASURE(0.001),#12805,
'DISTANCE_ACCURACY_VALUE',
'Maximum model space distance between geometric entities at asserted c
onnectivities');
#12786=(
GEOMETRIC_REPRESENTATION_CONTEXT(3)
GLOBAL_UNCERTAINTY_ASSIGNED_CONTEXT((#12750))
GLOBAL_UNIT_ASSIGNED_CONTEXT((#12805,#12807,#12808))
REPRESENTATION_CONTEXT('','3D')
);
#12804=(
GEOMETRIC_REPRESENTATION_CONTEXT(3)
GLOBAL_UNCERTAINTY_ASSIGNED_CONTEXT((#12768))
GLOBAL_UNIT_ASSIGNED_CONTEXT((#12805,#12807,#12808))
REPRESENTATION_CONTEXT('','3D')
);
#12805=(
LENGTH_UNIT()
NAMED_UNIT(*)
SI_UNIT(.CENTI.,.METRE.)
);
#12807=(
NAMED_UNIT(*)
PLANE_ANGLE_UNIT()
SI_UNIT($,.RADIAN.)
);
#12808=(
NAMED_UNIT(*)
SI_UNIT($,.STERADIAN.)
SOLID_ANGLE_UNIT()
);
#12826=SHAPE_DEFINITION_REPRESENTATION(#12861,#13016);
#12861=PRODUCT_DEFINITION_SHAPE('',$,#13052);
#13016=SHAPE_REPRESENTATION('',(#7995),#12786);
#13034=PRODUCT_DEFINITION_CONTEXT('part definition',#13141,'design');
#13052=PRODUCT_DEFINITION('Linear Guide Rail - 15 mm, 220 mm Long',
'Linear Guide Rail - 15 mm, 220 mm Long',#13087,#13034);
#13087=PRODUCT_DEFINITION_FORMATION('',$,#13160);
#13141=APPLICATION_CONTEXT(
'Core Data for Automotive Mechanical Design Process');
#13142=PRODUCT_CONTEXT('part definition',#13141,'mechanical');
#13160=PRODUCT('Linear Guide Rail - 15 mm, 220 mm Long',
'Linear Guide Rail - 15 mm, 220 mm Long',
'Linear Guide Rail - 15 mm, 220 mm Long',(#13142));
#13234=COLOUR_RGB('Sky Blue',0.24,0.69,0.87);
#13235=FILL_AREA_STYLE_COLOUR('',#13234);
#13236=FILL_AREA_STYLE('',(#13235));
#13237=SURFACE_STYLE_FILL_AREA(#13236);
#13238=SURFACE_SIDE_STYLE('',(#13237));
#13239=SURFACE_STYLE_USAGE(.BOTH.,#13238);
#13240=PRESENTATION_STYLE_ASSIGNMENT((#13239));
ENDSEC;
END-ISO-10303-21;
